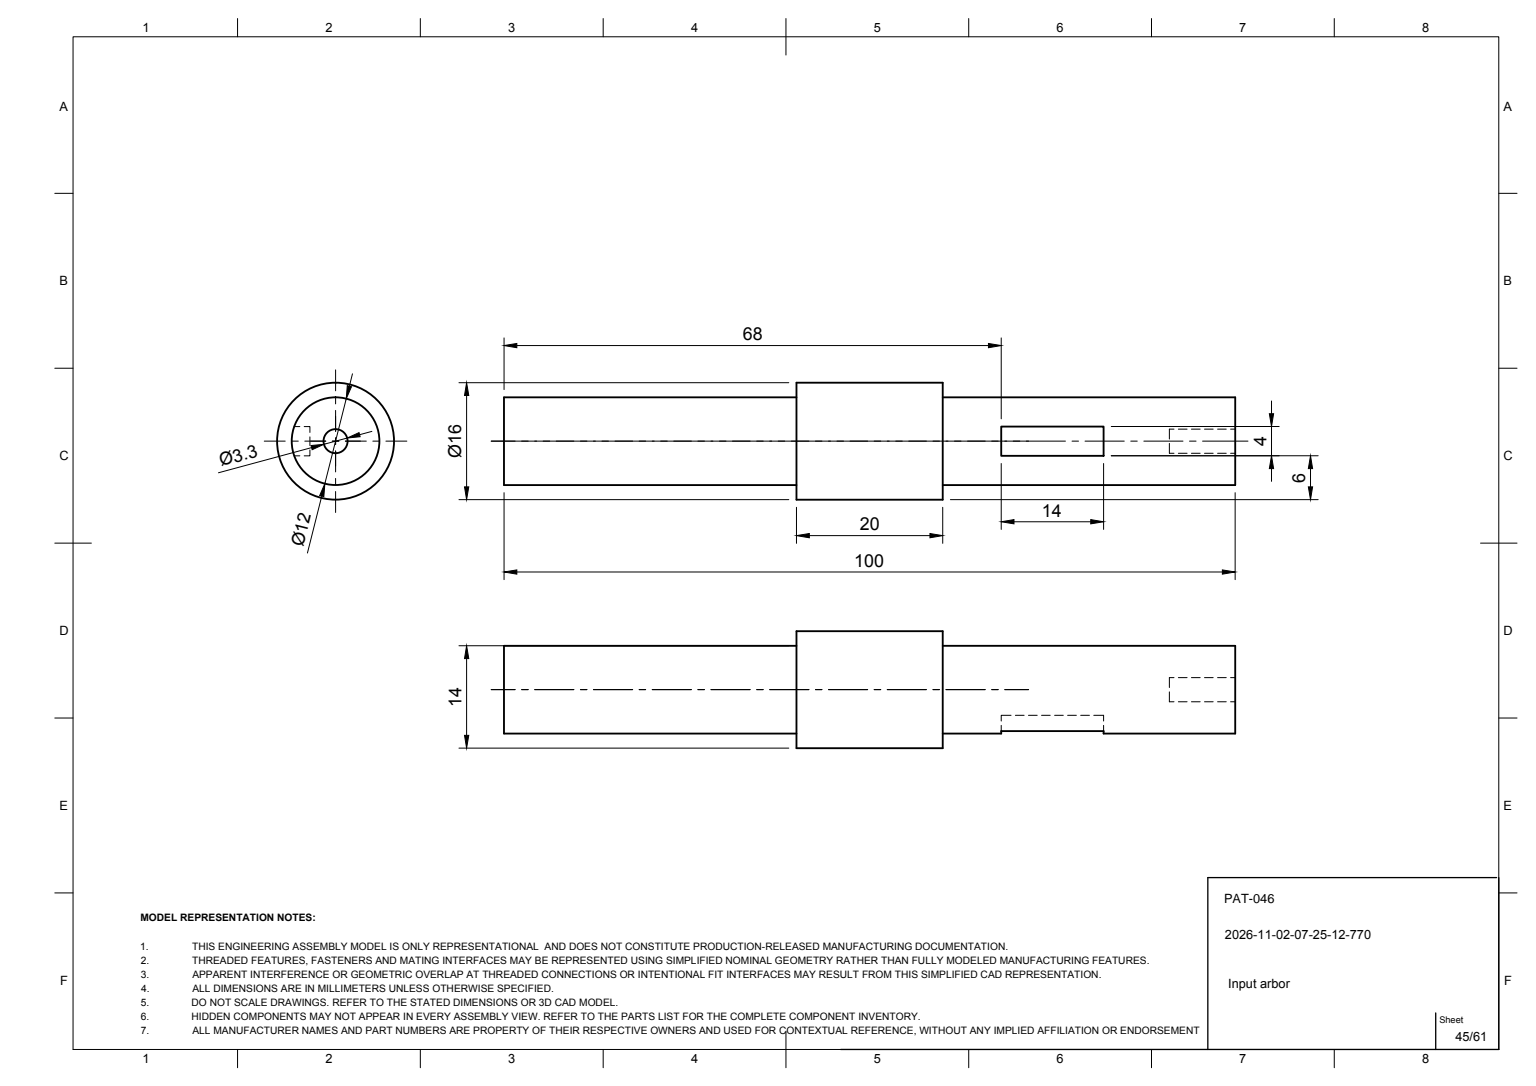
ISO-10303-21;
HEADER;
/* Generated by software containing ST-Developer
 * from STEP Tools, Inc. (www.steptools.com) 
 */

FILE_DESCRIPTION(
/* description */ ('Gear mesh backlash fixture'),
/* implementation_level */ '2;1');

FILE_NAME(
/* name */ 'Input arbor.step',
/* time_stamp */ '2026-10-28T03:26:00-07:00',
/* author */ (''),
/* organization */ (''),
/* preprocessor_version */ 'ST-DEVELOPER v20.2',
/* originating_system */ 'Autodesk Translation Framework v15.17.0.0',
/* authorisation */ '');

FILE_SCHEMA (('AUTOMOTIVE_DESIGN { 1 0 10303 214 3 1 1 }'));
ENDSEC;

DATA;
#10=MECHANICAL_DESIGN_GEOMETRIC_PRESENTATION_REPRESENTATION('',(#1064),#57900);
#949=SHAPE_REPRESENTATION_RELATIONSHIP('SRR','None',#58149,#999);
#999=ADVANCED_BREP_SHAPE_REPRESENTATION('',(#1127),#57882);
#1064=STYLED_ITEM('',(#58451),#1127);
#1127=MANIFOLD_SOLID_BREP('Body1',#13626);
#1291=FACE_BOUND('',#3016,.T.);
#1292=FACE_BOUND('',#3018,.T.);
#1293=FACE_BOUND('',#3022,.T.);
#1294=FACE_BOUND('',#3024,.T.);
#1549=PLANE('',#15046);
#1550=PLANE('',#15047);
#1551=PLANE('',#15048);
#1552=PLANE('',#15050);
#1553=PLANE('',#15051);
#1554=PLANE('',#15052);
#1555=PLANE('',#15054);
#1556=PLANE('',#15057);
#1557=PLANE('',#15065);
#1558=PLANE('',#15066);
#2095=FACE_OUTER_BOUND('',#3008,.T.);
#2096=FACE_OUTER_BOUND('',#3009,.T.);
#2097=FACE_OUTER_BOUND('',#3010,.T.);
#2098=FACE_OUTER_BOUND('',#3011,.T.);
#2099=FACE_OUTER_BOUND('',#3012,.T.);
#2100=FACE_OUTER_BOUND('',#3013,.T.);
#2101=FACE_OUTER_BOUND('',#3014,.T.);
#2102=FACE_OUTER_BOUND('',#3015,.T.);
#2103=FACE_OUTER_BOUND('',#3017,.T.);
#2104=FACE_OUTER_BOUND('',#3019,.T.);
#2105=FACE_OUTER_BOUND('',#3020,.T.);
#2106=FACE_OUTER_BOUND('',#3021,.T.);
#2107=FACE_OUTER_BOUND('',#3023,.T.);
#2108=FACE_OUTER_BOUND('',#3025,.T.);
#3008=EDGE_LOOP('',(#10687,#10688,#10689,#10690));
#3009=EDGE_LOOP('',(#10691));
#3010=EDGE_LOOP('',(#10692,#10693,#10694,#10695));
#3011=EDGE_LOOP('',(#10696,#10697,#10698,#10699));
#3012=EDGE_LOOP('',(#10700,#10701,#10702,#10703));
#3013=EDGE_LOOP('',(#10704,#10705,#10706,#10707));
#3014=EDGE_LOOP('',(#10708,#10709,#10710,#10711));
#3015=EDGE_LOOP('',(#10712));
#3016=EDGE_LOOP('',(#10713));
#3017=EDGE_LOOP('',(#10714));
#3018=EDGE_LOOP('',(#10715));
#3019=EDGE_LOOP('',(#10716,#10717,#10718,#10719));
#3020=EDGE_LOOP('',(#10720,#10721,#10722,#10723));
#3021=EDGE_LOOP('',(#10724,#10725,#10726,#10727));
#3022=EDGE_LOOP('',(#10728,#10729,#10730,#10731));
#3023=EDGE_LOOP('',(#10732));
#3024=EDGE_LOOP('',(#10733));
#3025=EDGE_LOOP('',(#10734));
#3879=LINE('',#22004,#4768);
#3880=LINE('',#22010,#4769);
#3881=LINE('',#22012,#4770);
#3882=LINE('',#22014,#4771);
#3883=LINE('',#22015,#4772);
#3884=LINE('',#22020,#4773);
#3885=LINE('',#22021,#4774);
#3886=LINE('',#22024,#4775);
#3887=LINE('',#22025,#4776);
#3888=LINE('',#22028,#4777);
#3889=LINE('',#22029,#4778);
#3890=LINE('',#22043,#4779);
#3891=LINE('',#22046,#4780);
#3892=LINE('',#22051,#4781);
#4768=VECTOR('',#17746,0.165);
#4769=VECTOR('',#17753,1.);
#4770=VECTOR('',#17754,1.);
#4771=VECTOR('',#17755,1.);
#4772=VECTOR('',#17756,1.);
#4773=VECTOR('',#17761,1.);
#4774=VECTOR('',#17762,1.);
#4775=VECTOR('',#17765,1.);
#4776=VECTOR('',#17766,1.);
#4777=VECTOR('',#17769,1.);
#4778=VECTOR('',#17770,1.);
#4779=VECTOR('',#17789,0.8);
#4780=VECTOR('',#17792,0.6);
#4781=VECTOR('',#17799,0.6);
#5582=CIRCLE('',#15044,0.165);
#5583=CIRCLE('',#15045,0.165);
#5584=CIRCLE('',#15049,0.6);
#5585=CIRCLE('',#15053,0.6);
#5586=CIRCLE('',#15055,0.8);
#5587=CIRCLE('',#15056,0.6);
#5588=CIRCLE('',#15058,0.8);
#5589=CIRCLE('',#15059,0.6);
#5590=CIRCLE('',#15062,0.6);
#5591=CIRCLE('',#15064,0.6);
#6394=VERTEX_POINT('',#22001);
#6395=VERTEX_POINT('',#22003);
#6396=VERTEX_POINT('',#22008);
#6397=VERTEX_POINT('',#22009);
#6398=VERTEX_POINT('',#22011);
#6399=VERTEX_POINT('',#22013);
#6400=VERTEX_POINT('',#22017);
#6401=VERTEX_POINT('',#22019);
#6402=VERTEX_POINT('',#22023);
#6403=VERTEX_POINT('',#22027);
#6404=VERTEX_POINT('',#22033);
#6405=VERTEX_POINT('',#22035);
#6406=VERTEX_POINT('',#22038);
#6407=VERTEX_POINT('',#22040);
#6408=VERTEX_POINT('',#22045);
#6409=VERTEX_POINT('',#22049);
#7930=EDGE_CURVE('',#6394,#6394,#5582,.T.);
#7931=EDGE_CURVE('',#6394,#6395,#3879,.T.);
#7932=EDGE_CURVE('',#6395,#6395,#5583,.T.);
#7933=EDGE_CURVE('',#6396,#6397,#3880,.T.);
#7934=EDGE_CURVE('',#6396,#6398,#3881,.T.);
#7935=EDGE_CURVE('',#6399,#6398,#3882,.T.);
#7936=EDGE_CURVE('',#6399,#6397,#3883,.T.);
#7937=EDGE_CURVE('',#6397,#6400,#5584,.T.);
#7938=EDGE_CURVE('',#6401,#6399,#3884,.T.);
#7939=EDGE_CURVE('',#6400,#6401,#3885,.T.);
#7940=EDGE_CURVE('',#6398,#6402,#3886,.T.);
#7941=EDGE_CURVE('',#6401,#6402,#3887,.T.);
#7942=EDGE_CURVE('',#6400,#6403,#3888,.T.);
#7943=EDGE_CURVE('',#6402,#6403,#3889,.T.);
#7944=EDGE_CURVE('',#6403,#6396,#5585,.T.);
#7945=EDGE_CURVE('',#6404,#6404,#5586,.T.);
#7946=EDGE_CURVE('',#6405,#6405,#5587,.T.);
#7947=EDGE_CURVE('',#6406,#6406,#5588,.T.);
#7948=EDGE_CURVE('',#6407,#6407,#5589,.T.);
#7949=EDGE_CURVE('',#6404,#6406,#3890,.T.);
#7950=EDGE_CURVE('',#6407,#6408,#3891,.T.);
#7951=EDGE_CURVE('',#6408,#6408,#5590,.T.);
#7952=EDGE_CURVE('',#6409,#6409,#5591,.T.);
#7953=EDGE_CURVE('',#6409,#6405,#3892,.T.);
#10687=ORIENTED_EDGE('',*,*,#7930,.F.);
#10688=ORIENTED_EDGE('',*,*,#7931,.T.);
#10689=ORIENTED_EDGE('',*,*,#7932,.F.);
#10690=ORIENTED_EDGE('',*,*,#7931,.F.);
#10691=ORIENTED_EDGE('',*,*,#7930,.T.);
#10692=ORIENTED_EDGE('',*,*,#7933,.F.);
#10693=ORIENTED_EDGE('',*,*,#7934,.T.);
#10694=ORIENTED_EDGE('',*,*,#7935,.F.);
#10695=ORIENTED_EDGE('',*,*,#7936,.T.);
#10696=ORIENTED_EDGE('',*,*,#7937,.F.);
#10697=ORIENTED_EDGE('',*,*,#7936,.F.);
#10698=ORIENTED_EDGE('',*,*,#7938,.F.);
#10699=ORIENTED_EDGE('',*,*,#7939,.F.);
#10700=ORIENTED_EDGE('',*,*,#7938,.T.);
#10701=ORIENTED_EDGE('',*,*,#7935,.T.);
#10702=ORIENTED_EDGE('',*,*,#7940,.T.);
#10703=ORIENTED_EDGE('',*,*,#7941,.F.);
#10704=ORIENTED_EDGE('',*,*,#7942,.F.);
#10705=ORIENTED_EDGE('',*,*,#7939,.T.);
#10706=ORIENTED_EDGE('',*,*,#7941,.T.);
#10707=ORIENTED_EDGE('',*,*,#7943,.T.);
#10708=ORIENTED_EDGE('',*,*,#7944,.F.);
#10709=ORIENTED_EDGE('',*,*,#7943,.F.);
#10710=ORIENTED_EDGE('',*,*,#7940,.F.);
#10711=ORIENTED_EDGE('',*,*,#7934,.F.);
#10712=ORIENTED_EDGE('',*,*,#7945,.T.);
#10713=ORIENTED_EDGE('',*,*,#7946,.F.);
#10714=ORIENTED_EDGE('',*,*,#7947,.F.);
#10715=ORIENTED_EDGE('',*,*,#7948,.F.);
#10716=ORIENTED_EDGE('',*,*,#7945,.F.);
#10717=ORIENTED_EDGE('',*,*,#7949,.T.);
#10718=ORIENTED_EDGE('',*,*,#7947,.T.);
#10719=ORIENTED_EDGE('',*,*,#7949,.F.);
#10720=ORIENTED_EDGE('',*,*,#7948,.T.);
#10721=ORIENTED_EDGE('',*,*,#7950,.T.);
#10722=ORIENTED_EDGE('',*,*,#7951,.T.);
#10723=ORIENTED_EDGE('',*,*,#7950,.F.);
#10724=ORIENTED_EDGE('',*,*,#7952,.F.);
#10725=ORIENTED_EDGE('',*,*,#7953,.T.);
#10726=ORIENTED_EDGE('',*,*,#7946,.T.);
#10727=ORIENTED_EDGE('',*,*,#7953,.F.);
#10728=ORIENTED_EDGE('',*,*,#7942,.T.);
#10729=ORIENTED_EDGE('',*,*,#7944,.T.);
#10730=ORIENTED_EDGE('',*,*,#7933,.T.);
#10731=ORIENTED_EDGE('',*,*,#7937,.T.);
#10732=ORIENTED_EDGE('',*,*,#7952,.T.);
#10733=ORIENTED_EDGE('',*,*,#7932,.T.);
#10734=ORIENTED_EDGE('',*,*,#7951,.F.);
#12716=CYLINDRICAL_SURFACE('',#15043,0.165);
#12717=CYLINDRICAL_SURFACE('',#15060,0.8);
#12718=CYLINDRICAL_SURFACE('',#15061,0.6);
#12719=CYLINDRICAL_SURFACE('',#15063,0.6);
#13212=ADVANCED_FACE('',(#2095),#12716,.F.);
#13213=ADVANCED_FACE('',(#2096),#1549,.T.);
#13214=ADVANCED_FACE('',(#2097),#1550,.F.);
#13215=ADVANCED_FACE('',(#2098),#1551,.T.);
#13216=ADVANCED_FACE('',(#2099),#1552,.F.);
#13217=ADVANCED_FACE('',(#2100),#1553,.F.);
#13218=ADVANCED_FACE('',(#2101),#1554,.F.);
#13219=ADVANCED_FACE('',(#2102,#1291),#1555,.T.);
#13220=ADVANCED_FACE('',(#2103,#1292),#1556,.F.);
#13221=ADVANCED_FACE('',(#2104),#12717,.T.);
#13222=ADVANCED_FACE('',(#2105),#12718,.T.);
#13223=ADVANCED_FACE('',(#2106,#1293),#12719,.T.);
#13224=ADVANCED_FACE('',(#2107,#1294),#1557,.T.);
#13225=ADVANCED_FACE('',(#2108),#1558,.F.);
#13626=CLOSED_SHELL('',(#13212,#13213,#13214,#13215,#13216,#13217,#13218,
#13219,#13220,#13221,#13222,#13223,#13224,#13225));
#15042=AXIS2_PLACEMENT_3D('',#21999,#17740,#17741);
#15043=AXIS2_PLACEMENT_3D('',#22000,#17742,#17743);
#15044=AXIS2_PLACEMENT_3D('',#22002,#17744,#17745);
#15045=AXIS2_PLACEMENT_3D('',#22005,#17747,#17748);
#15046=AXIS2_PLACEMENT_3D('',#22006,#17749,#17750);
#15047=AXIS2_PLACEMENT_3D('',#22007,#17751,#17752);
#15048=AXIS2_PLACEMENT_3D('',#22016,#17757,#17758);
#15049=AXIS2_PLACEMENT_3D('',#22018,#17759,#17760);
#15050=AXIS2_PLACEMENT_3D('',#22022,#17763,#17764);
#15051=AXIS2_PLACEMENT_3D('',#22026,#17767,#17768);
#15052=AXIS2_PLACEMENT_3D('',#22030,#17771,#17772);
#15053=AXIS2_PLACEMENT_3D('',#22031,#17773,#17774);
#15054=AXIS2_PLACEMENT_3D('',#22032,#17775,#17776);
#15055=AXIS2_PLACEMENT_3D('',#22034,#17777,#17778);
#15056=AXIS2_PLACEMENT_3D('',#22036,#17779,#17780);
#15057=AXIS2_PLACEMENT_3D('',#22037,#17781,#17782);
#15058=AXIS2_PLACEMENT_3D('',#22039,#17783,#17784);
#15059=AXIS2_PLACEMENT_3D('',#22041,#17785,#17786);
#15060=AXIS2_PLACEMENT_3D('',#22042,#17787,#17788);
#15061=AXIS2_PLACEMENT_3D('',#22044,#17790,#17791);
#15062=AXIS2_PLACEMENT_3D('',#22047,#17793,#17794);
#15063=AXIS2_PLACEMENT_3D('',#22048,#17795,#17796);
#15064=AXIS2_PLACEMENT_3D('',#22050,#17797,#17798);
#15065=AXIS2_PLACEMENT_3D('',#22052,#17800,#17801);
#15066=AXIS2_PLACEMENT_3D('',#22053,#17802,#17803);
#17740=DIRECTION('axis',(0.,0.,1.));
#17741=DIRECTION('refdir',(1.,0.,0.));
#17742=DIRECTION('center_axis',(0.,0.,1.));
#17743=DIRECTION('ref_axis',(1.,0.,0.));
#17744=DIRECTION('center_axis',(0.,0.,1.));
#17745=DIRECTION('ref_axis',(1.,0.,0.));
#17746=DIRECTION('',(0.,0.,1.));
#17747=DIRECTION('center_axis',(0.,0.,-1.));
#17748=DIRECTION('ref_axis',(1.,0.,0.));
#17749=DIRECTION('center_axis',(0.,0.,1.));
#17750=DIRECTION('ref_axis',(1.,0.,0.));
#17751=DIRECTION('center_axis',(-1.,0.,0.));
#17752=DIRECTION('ref_axis',(0.,-1.,0.));
#17753=DIRECTION('',(0.,0.,-1.));
#17754=DIRECTION('',(0.,-1.,0.));
#17755=DIRECTION('',(0.,0.,1.));
#17756=DIRECTION('',(0.,1.,0.));
#17757=DIRECTION('center_axis',(0.,0.,1.));
#17758=DIRECTION('ref_axis',(1.,0.,0.));
#17759=DIRECTION('center_axis',(0.,0.,-1.));
#17760=DIRECTION('ref_axis',(1.,0.,0.));
#17761=DIRECTION('',(-1.,0.,0.));
#17762=DIRECTION('',(0.,-1.,0.));
#17763=DIRECTION('center_axis',(0.,-1.,0.));
#17764=DIRECTION('ref_axis',(1.,0.,0.));
#17765=DIRECTION('',(1.,0.,0.));
#17766=DIRECTION('',(0.,0.,1.));
#17767=DIRECTION('center_axis',(1.,0.,0.));
#17768=DIRECTION('ref_axis',(0.,1.,0.));
#17769=DIRECTION('',(0.,0.,1.));
#17770=DIRECTION('',(0.,1.,0.));
#17771=DIRECTION('center_axis',(0.,0.,1.));
#17772=DIRECTION('ref_axis',(1.,0.,0.));
#17773=DIRECTION('center_axis',(0.,0.,1.));
#17774=DIRECTION('ref_axis',(1.,0.,0.));
#17775=DIRECTION('center_axis',(0.,0.,1.));
#17776=DIRECTION('ref_axis',(1.,0.,0.));
#17777=DIRECTION('center_axis',(0.,0.,1.));
#17778=DIRECTION('ref_axis',(1.,0.,0.));
#17779=DIRECTION('center_axis',(0.,0.,1.));
#17780=DIRECTION('ref_axis',(1.,0.,0.));
#17781=DIRECTION('center_axis',(0.,0.,1.));
#17782=DIRECTION('ref_axis',(1.,0.,0.));
#17783=DIRECTION('center_axis',(0.,0.,1.));
#17784=DIRECTION('ref_axis',(1.,0.,0.));
#17785=DIRECTION('center_axis',(0.,0.,-1.));
#17786=DIRECTION('ref_axis',(1.,0.,0.));
#17787=DIRECTION('center_axis',(0.,0.,1.));
#17788=DIRECTION('ref_axis',(1.,0.,0.));
#17789=DIRECTION('',(0.,0.,-1.));
#17790=DIRECTION('center_axis',(0.,0.,1.));
#17791=DIRECTION('ref_axis',(1.,0.,0.));
#17792=DIRECTION('',(0.,0.,-1.));
#17793=DIRECTION('center_axis',(0.,0.,1.));
#17794=DIRECTION('ref_axis',(1.,0.,0.));
#17795=DIRECTION('center_axis',(0.,0.,1.));
#17796=DIRECTION('ref_axis',(1.,0.,0.));
#17797=DIRECTION('center_axis',(0.,0.,1.));
#17798=DIRECTION('ref_axis',(1.,0.,0.));
#17799=DIRECTION('',(0.,0.,-1.));
#17800=DIRECTION('center_axis',(0.,0.,1.));
#17801=DIRECTION('ref_axis',(1.,0.,0.));
#17802=DIRECTION('center_axis',(0.,0.,1.));
#17803=DIRECTION('ref_axis',(1.,0.,0.));
#21999=CARTESIAN_POINT('',(0.,0.,0.));
#22000=CARTESIAN_POINT('Origin',(0.,0.,14.1));
#22001=CARTESIAN_POINT('',(-0.165,-2.02066721859313E-17,14.1));
#22002=CARTESIAN_POINT('Origin',(0.,0.,14.1));
#22003=CARTESIAN_POINT('',(-0.165,2.02066721859313E-17,15.));
#22004=CARTESIAN_POINT('',(-0.165,-2.02066721859313E-17,14.1));
#22005=CARTESIAN_POINT('Origin',(0.,0.,15.));
#22006=CARTESIAN_POINT('Origin',(0.,0.,14.1));
#22007=CARTESIAN_POINT('Origin',(-0.2,0.7,11.8));
#22008=CARTESIAN_POINT('',(-0.2,0.565685424949238,13.2));
#22009=CARTESIAN_POINT('',(-0.2,0.565685424949238,11.8));
#22010=CARTESIAN_POINT('',(-0.2,0.565685424949238,5.));
#22011=CARTESIAN_POINT('',(-0.2,0.35,13.2));
#22012=CARTESIAN_POINT('',(-0.2,0.35,13.2));
#22013=CARTESIAN_POINT('',(-0.2,0.35,11.8));
#22014=CARTESIAN_POINT('',(-0.2,0.35,11.8));
#22015=CARTESIAN_POINT('',(-0.2,0.35,11.8));
#22016=CARTESIAN_POINT('Origin',(0.,0.525,11.8));
#22017=CARTESIAN_POINT('',(0.2,0.565685424949238,11.8));
#22018=CARTESIAN_POINT('Origin',(0.,0.,11.8));
#22019=CARTESIAN_POINT('',(0.2,0.35,11.8));
#22020=CARTESIAN_POINT('',(0.2,0.35,11.8));
#22021=CARTESIAN_POINT('',(0.2,0.7,11.8));
#22022=CARTESIAN_POINT('Origin',(-0.2,0.35,11.8));
#22023=CARTESIAN_POINT('',(0.2,0.35,13.2));
#22024=CARTESIAN_POINT('',(0.2,0.35,13.2));
#22025=CARTESIAN_POINT('',(0.2,0.35,11.8));
#22026=CARTESIAN_POINT('Origin',(0.2,0.35,11.8));
#22027=CARTESIAN_POINT('',(0.2,0.565685424949238,13.2));
#22028=CARTESIAN_POINT('',(0.2,0.565685424949238,5.));
#22029=CARTESIAN_POINT('',(0.2,0.7,13.2));
#22030=CARTESIAN_POINT('Origin',(0.,0.525,13.2));
#22031=CARTESIAN_POINT('Origin',(0.,0.,13.2));
#22032=CARTESIAN_POINT('Origin',(0.,0.,11.));
#22033=CARTESIAN_POINT('',(-0.8,-9.79717439317883E-17,11.));
#22034=CARTESIAN_POINT('Origin',(0.,0.,11.));
#22035=CARTESIAN_POINT('',(-0.6,-7.34788079488412E-17,11.));
#22036=CARTESIAN_POINT('Origin',(0.,0.,11.));
#22037=CARTESIAN_POINT('Origin',(0.,0.,9.));
#22038=CARTESIAN_POINT('',(-0.8,-9.79717439317883E-17,9.));
#22039=CARTESIAN_POINT('Origin',(0.,0.,9.));
#22040=CARTESIAN_POINT('',(-0.6,7.34788079488412E-17,9.));
#22041=CARTESIAN_POINT('Origin',(0.,0.,9.));
#22042=CARTESIAN_POINT('Origin',(0.,0.,9.));
#22043=CARTESIAN_POINT('',(-0.8,-9.79717439317883E-17,9.));
#22044=CARTESIAN_POINT('Origin',(0.,0.,5.));
#22045=CARTESIAN_POINT('',(-0.6,-7.34788079488412E-17,5.));
#22046=CARTESIAN_POINT('',(-0.6,-7.34788079488412E-17,5.));
#22047=CARTESIAN_POINT('Origin',(0.,0.,5.));
#22048=CARTESIAN_POINT('Origin',(0.,0.,5.));
#22049=CARTESIAN_POINT('',(-0.6,-7.34788079488412E-17,15.));
#22050=CARTESIAN_POINT('Origin',(0.,0.,15.));
#22051=CARTESIAN_POINT('',(-0.6,-7.34788079488412E-17,5.));
#22052=CARTESIAN_POINT('Origin',(0.,0.,15.));
#22053=CARTESIAN_POINT('Origin',(0.,0.,5.));
#57823=UNCERTAINTY_MEASURE_WITH_UNIT(LENGTH_MEASURE(0.001),#57901,
'DISTANCE_ACCURACY_VALUE',
'Maximum model space distance between geometric entities at asserted c
onnectivities');
#57841=UNCERTAINTY_MEASURE_WITH_UNIT(LENGTH_MEASURE(0.001),#57901,
'DISTANCE_ACCURACY_VALUE',
'Maximum model space distance between geometric entities at asserted c
onnectivities');
#57882=(
GEOMETRIC_REPRESENTATION_CONTEXT(3)
GLOBAL_UNCERTAINTY_ASSIGNED_CONTEXT((#57823))
GLOBAL_UNIT_ASSIGNED_CONTEXT((#57901,#57903,#57904))
REPRESENTATION_CONTEXT('','3D')
);
#57900=(
GEOMETRIC_REPRESENTATION_CONTEXT(3)
GLOBAL_UNCERTAINTY_ASSIGNED_CONTEXT((#57841))
GLOBAL_UNIT_ASSIGNED_CONTEXT((#57901,#57903,#57904))
REPRESENTATION_CONTEXT('','3D')
);
#57901=(
LENGTH_UNIT()
NAMED_UNIT(*)
SI_UNIT(.CENTI.,.METRE.)
);
#57903=(
NAMED_UNIT(*)
PLANE_ANGLE_UNIT()
SI_UNIT($,.RADIAN.)
);
#57904=(
NAMED_UNIT(*)
SI_UNIT($,.STERADIAN.)
SOLID_ANGLE_UNIT()
);
#57945=SHAPE_DEFINITION_REPRESENTATION(#58016,#58149);
#58016=PRODUCT_DEFINITION_SHAPE('',$,#58208);
#58149=SHAPE_REPRESENTATION('',(#15042),#57882);
#58167=PRODUCT_DEFINITION_CONTEXT('part definition',#58343,'design');
#58208=PRODUCT_DEFINITION('Input arbor','Input arbor',#58266,#58167);
#58266=PRODUCT_DEFINITION_FORMATION('',$,#58385);
#58343=APPLICATION_CONTEXT(
'Core Data for Automotive Mechanical Design Process');
#58344=PRODUCT_CONTEXT('part definition',#58343,'mechanical');
#58385=PRODUCT('Input arbor','Input arbor','Input arbor',(#58344));
#58445=COLOUR_RGB('Light Blue',0.38,0.62,0.78);
#58446=FILL_AREA_STYLE_COLOUR('',#58445);
#58447=FILL_AREA_STYLE('',(#58446));
#58448=SURFACE_STYLE_FILL_AREA(#58447);
#58449=SURFACE_SIDE_STYLE('',(#58448));
#58450=SURFACE_STYLE_USAGE(.BOTH.,#58449);
#58451=PRESENTATION_STYLE_ASSIGNMENT((#58450));
ENDSEC;
END-ISO-10303-21;
